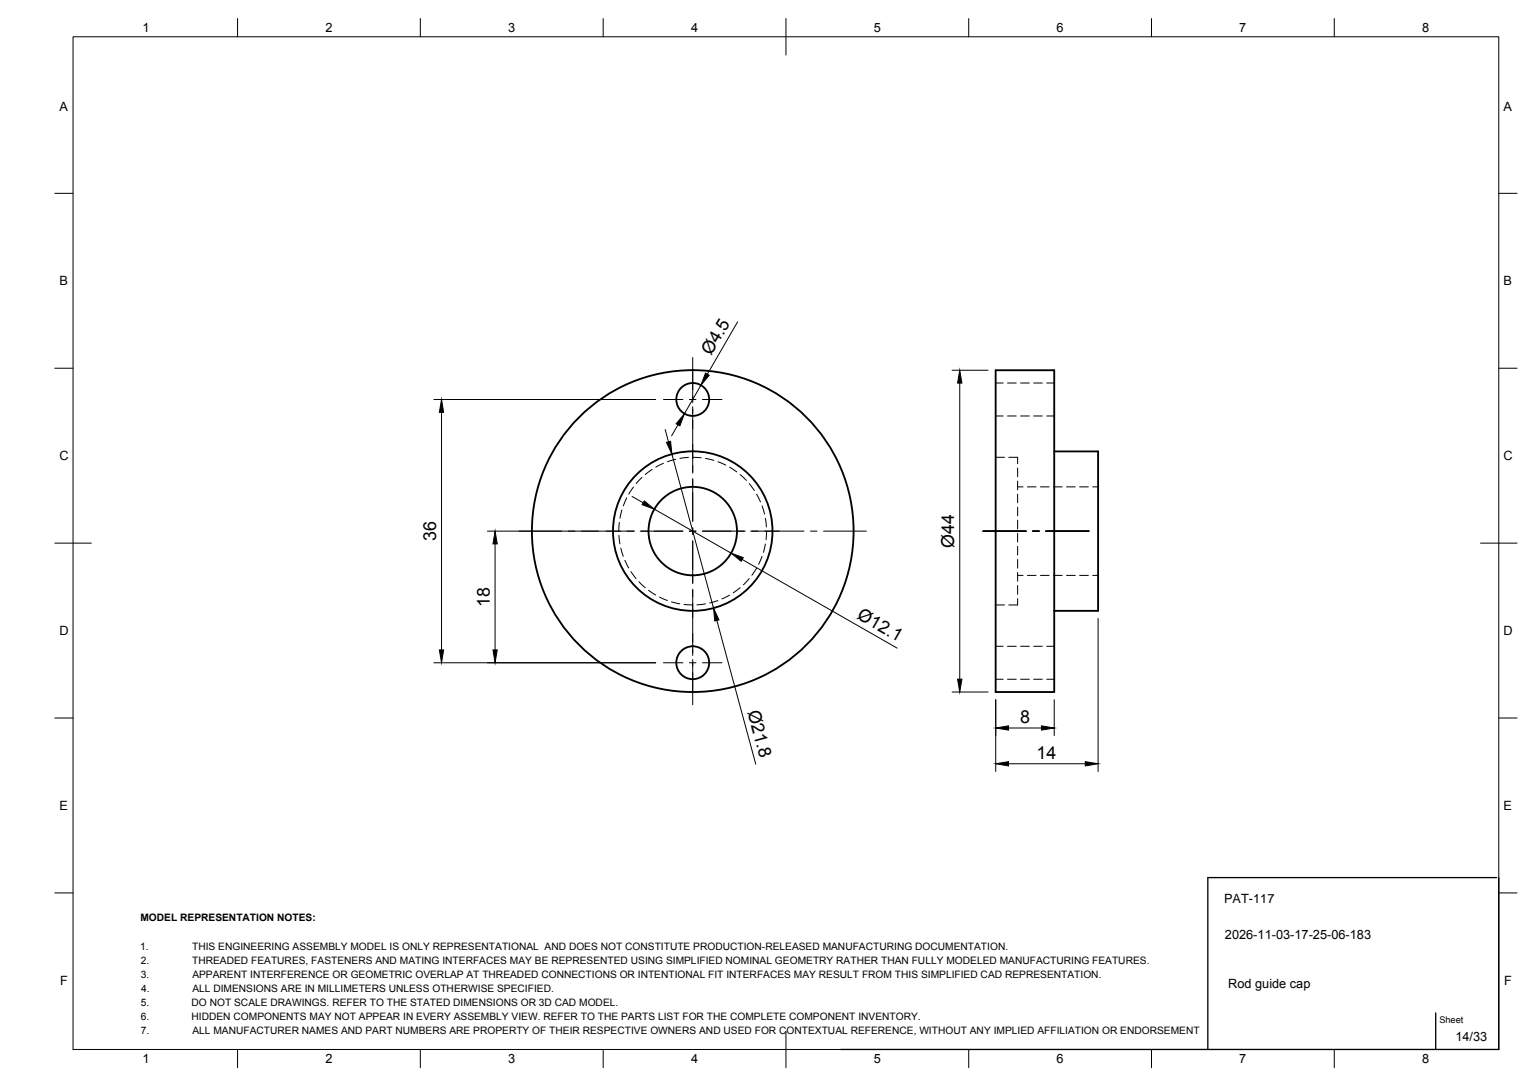
ISO-10303-21;
HEADER;
/* Generated by software containing ST-Developer
 * from STEP Tools, Inc. (www.steptools.com) 
 */

FILE_DESCRIPTION(
/* description */ ('Counterbalanced vertical column'),
/* implementation_level */ '2;1');

FILE_NAME(
/* name */ 'Rod guide cap.step',
/* time_stamp */ '2026-10-29T16:47:22-07:00',
/* author */ (''),
/* organization */ (''),
/* preprocessor_version */ 'ST-DEVELOPER v20.2',
/* originating_system */ 'Autodesk Translation Framework v15.17.0.0',
/* authorisation */ '');

FILE_SCHEMA (('AUTOMOTIVE_DESIGN { 1 0 10303 214 3 1 1 }'));
ENDSEC;

DATA;
#10=MECHANICAL_DESIGN_GEOMETRIC_PRESENTATION_REPRESENTATION('',(#359),#15040);
#289=SHAPE_REPRESENTATION_RELATIONSHIP('SRR','None',#15193,#324);
#324=ADVANCED_BREP_SHAPE_REPRESENTATION('',(#394),#15012);
#359=STYLED_ITEM('',(#15457),#394);
#394=MANIFOLD_SOLID_BREP('Body1',#7082);
#452=FACE_BOUND('',#1350,.T.);
#453=FACE_BOUND('',#1353,.T.);
#454=FACE_BOUND('',#1357,.T.);
#455=FACE_BOUND('',#1358,.T.);
#456=FACE_BOUND('',#1359,.T.);
#457=FACE_BOUND('',#1361,.T.);
#458=FACE_BOUND('',#1362,.T.);
#459=FACE_BOUND('',#1363,.T.);
#587=PLANE('',#7644);
#588=PLANE('',#7649);
#589=PLANE('',#7655);
#590=PLANE('',#7656);
#905=FACE_OUTER_BOUND('',#1346,.T.);
#906=FACE_OUTER_BOUND('',#1347,.T.);
#907=FACE_OUTER_BOUND('',#1348,.T.);
#908=FACE_OUTER_BOUND('',#1349,.T.);
#909=FACE_OUTER_BOUND('',#1351,.T.);
#910=FACE_OUTER_BOUND('',#1352,.T.);
#911=FACE_OUTER_BOUND('',#1354,.T.);
#912=FACE_OUTER_BOUND('',#1355,.T.);
#913=FACE_OUTER_BOUND('',#1356,.T.);
#914=FACE_OUTER_BOUND('',#1360,.T.);
#1346=EDGE_LOOP('',(#5118,#5119,#5120,#5121));
#1347=EDGE_LOOP('',(#5122,#5123,#5124,#5125));
#1348=EDGE_LOOP('',(#5126,#5127,#5128,#5129));
#1349=EDGE_LOOP('',(#5130));
#1350=EDGE_LOOP('',(#5131));
#1351=EDGE_LOOP('',(#5132,#5133,#5134,#5135));
#1352=EDGE_LOOP('',(#5136));
#1353=EDGE_LOOP('',(#5137));
#1354=EDGE_LOOP('',(#5138,#5139,#5140,#5141));
#1355=EDGE_LOOP('',(#5142,#5143,#5144,#5145));
#1356=EDGE_LOOP('',(#5146));
#1357=EDGE_LOOP('',(#5147));
#1358=EDGE_LOOP('',(#5148));
#1359=EDGE_LOOP('',(#5149));
#1360=EDGE_LOOP('',(#5150));
#1361=EDGE_LOOP('',(#5151));
#1362=EDGE_LOOP('',(#5152));
#1363=EDGE_LOOP('',(#5153));
#1870=LINE('',#10708,#2541);
#1871=LINE('',#10714,#2542);
#1872=LINE('',#10720,#2543);
#1873=LINE('',#10729,#2544);
#1874=LINE('',#10735,#2545);
#1875=LINE('',#10740,#2546);
#2541=VECTOR('',#8618,0.225);
#2542=VECTOR('',#8625,0.225);
#2543=VECTOR('',#8632,1.01);
#2544=VECTOR('',#8643,1.09);
#2545=VECTOR('',#8652,0.605);
#2546=VECTOR('',#8657,2.2);
#3139=CIRCLE('',#7636,0.225);
#3140=CIRCLE('',#7637,0.225);
#3141=CIRCLE('',#7639,0.225);
#3142=CIRCLE('',#7640,0.225);
#3143=CIRCLE('',#7642,1.01);
#3144=CIRCLE('',#7643,1.01);
#3145=CIRCLE('',#7645,0.605);
#3146=CIRCLE('',#7647,1.09);
#3147=CIRCLE('',#7648,1.09);
#3148=CIRCLE('',#7650,0.605);
#3149=CIRCLE('',#7653,2.2);
#3150=CIRCLE('',#7654,2.2);
#3416=VERTEX_POINT('',#10705);
#3417=VERTEX_POINT('',#10707);
#3418=VERTEX_POINT('',#10711);
#3419=VERTEX_POINT('',#10713);
#3420=VERTEX_POINT('',#10717);
#3421=VERTEX_POINT('',#10719);
#3422=VERTEX_POINT('',#10723);
#3423=VERTEX_POINT('',#10726);
#3424=VERTEX_POINT('',#10728);
#3425=VERTEX_POINT('',#10732);
#3426=VERTEX_POINT('',#10737);
#3427=VERTEX_POINT('',#10739);
#4060=EDGE_CURVE('',#3416,#3416,#3139,.T.);
#4061=EDGE_CURVE('',#3416,#3417,#1870,.T.);
#4062=EDGE_CURVE('',#3417,#3417,#3140,.T.);
#4063=EDGE_CURVE('',#3418,#3418,#3141,.T.);
#4064=EDGE_CURVE('',#3418,#3419,#1871,.T.);
#4065=EDGE_CURVE('',#3419,#3419,#3142,.T.);
#4066=EDGE_CURVE('',#3420,#3420,#3143,.T.);
#4067=EDGE_CURVE('',#3420,#3421,#1872,.T.);
#4068=EDGE_CURVE('',#3421,#3421,#3144,.T.);
#4069=EDGE_CURVE('',#3422,#3422,#3145,.T.);
#4070=EDGE_CURVE('',#3423,#3423,#3146,.T.);
#4071=EDGE_CURVE('',#3423,#3424,#1873,.T.);
#4072=EDGE_CURVE('',#3424,#3424,#3147,.T.);
#4073=EDGE_CURVE('',#3425,#3425,#3148,.T.);
#4074=EDGE_CURVE('',#3422,#3425,#1874,.T.);
#4075=EDGE_CURVE('',#3426,#3426,#3149,.T.);
#4076=EDGE_CURVE('',#3426,#3427,#1875,.T.);
#4077=EDGE_CURVE('',#3427,#3427,#3150,.T.);
#5118=ORIENTED_EDGE('',*,*,#4060,.F.);
#5119=ORIENTED_EDGE('',*,*,#4061,.T.);
#5120=ORIENTED_EDGE('',*,*,#4062,.F.);
#5121=ORIENTED_EDGE('',*,*,#4061,.F.);
#5122=ORIENTED_EDGE('',*,*,#4063,.F.);
#5123=ORIENTED_EDGE('',*,*,#4064,.T.);
#5124=ORIENTED_EDGE('',*,*,#4065,.F.);
#5125=ORIENTED_EDGE('',*,*,#4064,.F.);
#5126=ORIENTED_EDGE('',*,*,#4066,.F.);
#5127=ORIENTED_EDGE('',*,*,#4067,.T.);
#5128=ORIENTED_EDGE('',*,*,#4068,.F.);
#5129=ORIENTED_EDGE('',*,*,#4067,.F.);
#5130=ORIENTED_EDGE('',*,*,#4066,.T.);
#5131=ORIENTED_EDGE('',*,*,#4069,.F.);
#5132=ORIENTED_EDGE('',*,*,#4070,.F.);
#5133=ORIENTED_EDGE('',*,*,#4071,.T.);
#5134=ORIENTED_EDGE('',*,*,#4072,.T.);
#5135=ORIENTED_EDGE('',*,*,#4071,.F.);
#5136=ORIENTED_EDGE('',*,*,#4072,.F.);
#5137=ORIENTED_EDGE('',*,*,#4073,.F.);
#5138=ORIENTED_EDGE('',*,*,#4069,.T.);
#5139=ORIENTED_EDGE('',*,*,#4074,.T.);
#5140=ORIENTED_EDGE('',*,*,#4073,.T.);
#5141=ORIENTED_EDGE('',*,*,#4074,.F.);
#5142=ORIENTED_EDGE('',*,*,#4075,.F.);
#5143=ORIENTED_EDGE('',*,*,#4076,.T.);
#5144=ORIENTED_EDGE('',*,*,#4077,.T.);
#5145=ORIENTED_EDGE('',*,*,#4076,.F.);
#5146=ORIENTED_EDGE('',*,*,#4075,.T.);
#5147=ORIENTED_EDGE('',*,*,#4062,.T.);
#5148=ORIENTED_EDGE('',*,*,#4065,.T.);
#5149=ORIENTED_EDGE('',*,*,#4068,.T.);
#5150=ORIENTED_EDGE('',*,*,#4077,.F.);
#5151=ORIENTED_EDGE('',*,*,#4060,.T.);
#5152=ORIENTED_EDGE('',*,*,#4063,.T.);
#5153=ORIENTED_EDGE('',*,*,#4070,.T.);
#6597=CYLINDRICAL_SURFACE('',#7635,0.225);
#6598=CYLINDRICAL_SURFACE('',#7638,0.225);
#6599=CYLINDRICAL_SURFACE('',#7641,1.01);
#6600=CYLINDRICAL_SURFACE('',#7646,1.09);
#6601=CYLINDRICAL_SURFACE('',#7651,0.605);
#6602=CYLINDRICAL_SURFACE('',#7652,2.2);
#6747=ADVANCED_FACE('',(#905),#6597,.F.);
#6748=ADVANCED_FACE('',(#906),#6598,.F.);
#6749=ADVANCED_FACE('',(#907),#6599,.F.);
#6750=ADVANCED_FACE('',(#908,#452),#587,.T.);
#6751=ADVANCED_FACE('',(#909),#6600,.T.);
#6752=ADVANCED_FACE('',(#910,#453),#588,.F.);
#6753=ADVANCED_FACE('',(#911),#6601,.F.);
#6754=ADVANCED_FACE('',(#912),#6602,.T.);
#6755=ADVANCED_FACE('',(#913,#454,#455,#456),#589,.T.);
#6756=ADVANCED_FACE('',(#914,#457,#458,#459),#590,.F.);
#7082=CLOSED_SHELL('',(#6747,#6748,#6749,#6750,#6751,#6752,#6753,#6754,
#6755,#6756));
#7634=AXIS2_PLACEMENT_3D('',#10703,#8612,#8613);
#7635=AXIS2_PLACEMENT_3D('',#10704,#8614,#8615);
#7636=AXIS2_PLACEMENT_3D('',#10706,#8616,#8617);
#7637=AXIS2_PLACEMENT_3D('',#10709,#8619,#8620);
#7638=AXIS2_PLACEMENT_3D('',#10710,#8621,#8622);
#7639=AXIS2_PLACEMENT_3D('',#10712,#8623,#8624);
#7640=AXIS2_PLACEMENT_3D('',#10715,#8626,#8627);
#7641=AXIS2_PLACEMENT_3D('',#10716,#8628,#8629);
#7642=AXIS2_PLACEMENT_3D('',#10718,#8630,#8631);
#7643=AXIS2_PLACEMENT_3D('',#10721,#8633,#8634);
#7644=AXIS2_PLACEMENT_3D('',#10722,#8635,#8636);
#7645=AXIS2_PLACEMENT_3D('',#10724,#8637,#8638);
#7646=AXIS2_PLACEMENT_3D('',#10725,#8639,#8640);
#7647=AXIS2_PLACEMENT_3D('',#10727,#8641,#8642);
#7648=AXIS2_PLACEMENT_3D('',#10730,#8644,#8645);
#7649=AXIS2_PLACEMENT_3D('',#10731,#8646,#8647);
#7650=AXIS2_PLACEMENT_3D('',#10733,#8648,#8649);
#7651=AXIS2_PLACEMENT_3D('',#10734,#8650,#8651);
#7652=AXIS2_PLACEMENT_3D('',#10736,#8653,#8654);
#7653=AXIS2_PLACEMENT_3D('',#10738,#8655,#8656);
#7654=AXIS2_PLACEMENT_3D('',#10741,#8658,#8659);
#7655=AXIS2_PLACEMENT_3D('',#10742,#8660,#8661);
#7656=AXIS2_PLACEMENT_3D('',#10743,#8662,#8663);
#8612=DIRECTION('axis',(0.,0.,1.));
#8613=DIRECTION('refdir',(1.,0.,0.));
#8614=DIRECTION('center_axis',(0.,0.,1.));
#8615=DIRECTION('ref_axis',(1.,0.,0.));
#8616=DIRECTION('center_axis',(0.,0.,1.));
#8617=DIRECTION('ref_axis',(1.,0.,0.));
#8618=DIRECTION('',(0.,0.,1.));
#8619=DIRECTION('center_axis',(0.,0.,-1.));
#8620=DIRECTION('ref_axis',(1.,0.,0.));
#8621=DIRECTION('center_axis',(0.,0.,1.));
#8622=DIRECTION('ref_axis',(1.,0.,0.));
#8623=DIRECTION('center_axis',(0.,0.,1.));
#8624=DIRECTION('ref_axis',(1.,0.,0.));
#8625=DIRECTION('',(0.,0.,1.));
#8626=DIRECTION('center_axis',(0.,0.,-1.));
#8627=DIRECTION('ref_axis',(1.,0.,0.));
#8628=DIRECTION('center_axis',(0.,0.,1.));
#8629=DIRECTION('ref_axis',(1.,0.,0.));
#8630=DIRECTION('center_axis',(0.,0.,1.));
#8631=DIRECTION('ref_axis',(1.,0.,0.));
#8632=DIRECTION('',(0.,0.,1.));
#8633=DIRECTION('center_axis',(0.,0.,-1.));
#8634=DIRECTION('ref_axis',(1.,0.,0.));
#8635=DIRECTION('center_axis',(0.,0.,1.));
#8636=DIRECTION('ref_axis',(1.,0.,0.));
#8637=DIRECTION('center_axis',(0.,0.,1.));
#8638=DIRECTION('ref_axis',(1.,0.,0.));
#8639=DIRECTION('center_axis',(0.,0.,1.));
#8640=DIRECTION('ref_axis',(1.,0.,0.));
#8641=DIRECTION('center_axis',(0.,0.,1.));
#8642=DIRECTION('ref_axis',(1.,0.,0.));
#8643=DIRECTION('',(0.,0.,-1.));
#8644=DIRECTION('center_axis',(0.,0.,1.));
#8645=DIRECTION('ref_axis',(1.,0.,0.));
#8646=DIRECTION('center_axis',(0.,0.,1.));
#8647=DIRECTION('ref_axis',(1.,0.,0.));
#8648=DIRECTION('center_axis',(0.,0.,-1.));
#8649=DIRECTION('ref_axis',(1.,0.,0.));
#8650=DIRECTION('center_axis',(0.,0.,1.));
#8651=DIRECTION('ref_axis',(1.,0.,0.));
#8652=DIRECTION('',(0.,0.,-1.));
#8653=DIRECTION('center_axis',(0.,0.,1.));
#8654=DIRECTION('ref_axis',(1.,0.,0.));
#8655=DIRECTION('center_axis',(0.,0.,1.));
#8656=DIRECTION('ref_axis',(1.,0.,0.));
#8657=DIRECTION('',(0.,0.,-1.));
#8658=DIRECTION('center_axis',(0.,0.,1.));
#8659=DIRECTION('ref_axis',(1.,0.,0.));
#8660=DIRECTION('center_axis',(0.,0.,1.));
#8661=DIRECTION('ref_axis',(1.,0.,0.));
#8662=DIRECTION('center_axis',(0.,0.,1.));
#8663=DIRECTION('ref_axis',(1.,0.,0.));
#10703=CARTESIAN_POINT('',(0.,0.,0.));
#10704=CARTESIAN_POINT('Origin',(-5.2,0.,19.9));
#10705=CARTESIAN_POINT('',(-5.425,-2.75545529808154E-17,20.));
#10706=CARTESIAN_POINT('Origin',(-5.2,0.,20.));
#10707=CARTESIAN_POINT('',(-5.425,2.75545529808154E-17,20.8));
#10708=CARTESIAN_POINT('',(-5.425,-2.75545529808154E-17,19.9));
#10709=CARTESIAN_POINT('Origin',(-5.2,0.,20.8));
#10710=CARTESIAN_POINT('Origin',(-8.8,0.,19.9));
#10711=CARTESIAN_POINT('',(-9.025,-2.75545529808154E-17,20.));
#10712=CARTESIAN_POINT('Origin',(-8.8,0.,20.));
#10713=CARTESIAN_POINT('',(-9.025,2.75545529808154E-17,20.8));
#10714=CARTESIAN_POINT('',(-9.025,-2.75545529808154E-17,19.9));
#10715=CARTESIAN_POINT('Origin',(-8.8,0.,20.8));
#10716=CARTESIAN_POINT('Origin',(-7.,0.,20.5));
#10717=CARTESIAN_POINT('',(-8.01,-1.23689326713883E-16,20.5));
#10718=CARTESIAN_POINT('Origin',(-7.,0.,20.5));
#10719=CARTESIAN_POINT('',(-8.01,1.23689326713883E-16,20.8));
#10720=CARTESIAN_POINT('',(-8.01,-1.23689326713883E-16,20.5));
#10721=CARTESIAN_POINT('Origin',(-7.,0.,20.8));
#10722=CARTESIAN_POINT('Origin',(-7.,0.,20.5));
#10723=CARTESIAN_POINT('',(-7.605,-7.40911313484149E-17,20.5));
#10724=CARTESIAN_POINT('Origin',(-7.,0.,20.5));
#10725=CARTESIAN_POINT('Origin',(-7.,0.,19.4));
#10726=CARTESIAN_POINT('',(-8.09,-1.33486501107061E-16,20.));
#10727=CARTESIAN_POINT('Origin',(-7.,0.,20.));
#10728=CARTESIAN_POINT('',(-8.09,-1.33486501107061E-16,19.4));
#10729=CARTESIAN_POINT('',(-8.09,-1.33486501107061E-16,19.4));
#10730=CARTESIAN_POINT('Origin',(-7.,0.,19.4));
#10731=CARTESIAN_POINT('Origin',(-7.,0.,19.4));
#10732=CARTESIAN_POINT('',(-7.605,-7.40911313484149E-17,19.4));
#10733=CARTESIAN_POINT('Origin',(-7.,0.,19.4));
#10734=CARTESIAN_POINT('Origin',(-7.,0.,20.));
#10735=CARTESIAN_POINT('',(-7.605,-7.40911313484149E-17,20.));
#10736=CARTESIAN_POINT('Origin',(-7.,0.,20.));
#10737=CARTESIAN_POINT('',(-9.2,-2.69422295812418E-16,20.8));
#10738=CARTESIAN_POINT('Origin',(-7.,0.,20.8));
#10739=CARTESIAN_POINT('',(-9.2,-2.69422295812418E-16,20.));
#10740=CARTESIAN_POINT('',(-9.2,-2.69422295812418E-16,20.));
#10741=CARTESIAN_POINT('Origin',(-7.,0.,20.));
#10742=CARTESIAN_POINT('Origin',(-7.,0.,20.8));
#10743=CARTESIAN_POINT('Origin',(-7.,0.,20.));
#14972=UNCERTAINTY_MEASURE_WITH_UNIT(LENGTH_MEASURE(0.001),#15041,
'DISTANCE_ACCURACY_VALUE',
'Maximum model space distance between geometric entities at asserted c
onnectivities');
#15000=UNCERTAINTY_MEASURE_WITH_UNIT(LENGTH_MEASURE(0.001),#15041,
'DISTANCE_ACCURACY_VALUE',
'Maximum model space distance between geometric entities at asserted c
onnectivities');
#15012=(
GEOMETRIC_REPRESENTATION_CONTEXT(3)
GLOBAL_UNCERTAINTY_ASSIGNED_CONTEXT((#14972))
GLOBAL_UNIT_ASSIGNED_CONTEXT((#15041,#15043,#15044))
REPRESENTATION_CONTEXT('','3D')
);
#15040=(
GEOMETRIC_REPRESENTATION_CONTEXT(3)
GLOBAL_UNCERTAINTY_ASSIGNED_CONTEXT((#15000))
GLOBAL_UNIT_ASSIGNED_CONTEXT((#15041,#15043,#15044))
REPRESENTATION_CONTEXT('','3D')
);
#15041=(
LENGTH_UNIT()
NAMED_UNIT(*)
SI_UNIT(.CENTI.,.METRE.)
);
#15043=(
NAMED_UNIT(*)
PLANE_ANGLE_UNIT()
SI_UNIT($,.RADIAN.)
);
#15044=(
NAMED_UNIT(*)
SI_UNIT($,.STERADIAN.)
SOLID_ANGLE_UNIT()
);
#15056=SHAPE_DEFINITION_REPRESENTATION(#15095,#15193);
#15095=PRODUCT_DEFINITION_SHAPE('',$,#15233);
#15193=SHAPE_REPRESENTATION('',(#7634),#15012);
#15221=PRODUCT_DEFINITION_CONTEXT('part definition',#15340,'design');
#15233=PRODUCT_DEFINITION('Rod guide cap','Rod guide cap',#15272,#15221);
#15272=PRODUCT_DEFINITION_FORMATION('',$,#15353);
#15340=APPLICATION_CONTEXT(
'Core Data for Automotive Mechanical Design Process');
#15341=PRODUCT_CONTEXT('part definition',#15340,'mechanical');
#15353=PRODUCT('Rod guide cap','Rod guide cap','Rod guide cap',(#15341));
#15451=COLOUR_RGB('Grey',0.48,0.52,0.57);
#15452=FILL_AREA_STYLE_COLOUR('',#15451);
#15453=FILL_AREA_STYLE('',(#15452));
#15454=SURFACE_STYLE_FILL_AREA(#15453);
#15455=SURFACE_SIDE_STYLE('',(#15454));
#15456=SURFACE_STYLE_USAGE(.BOTH.,#15455);
#15457=PRESENTATION_STYLE_ASSIGNMENT((#15456));
ENDSEC;
END-ISO-10303-21;
